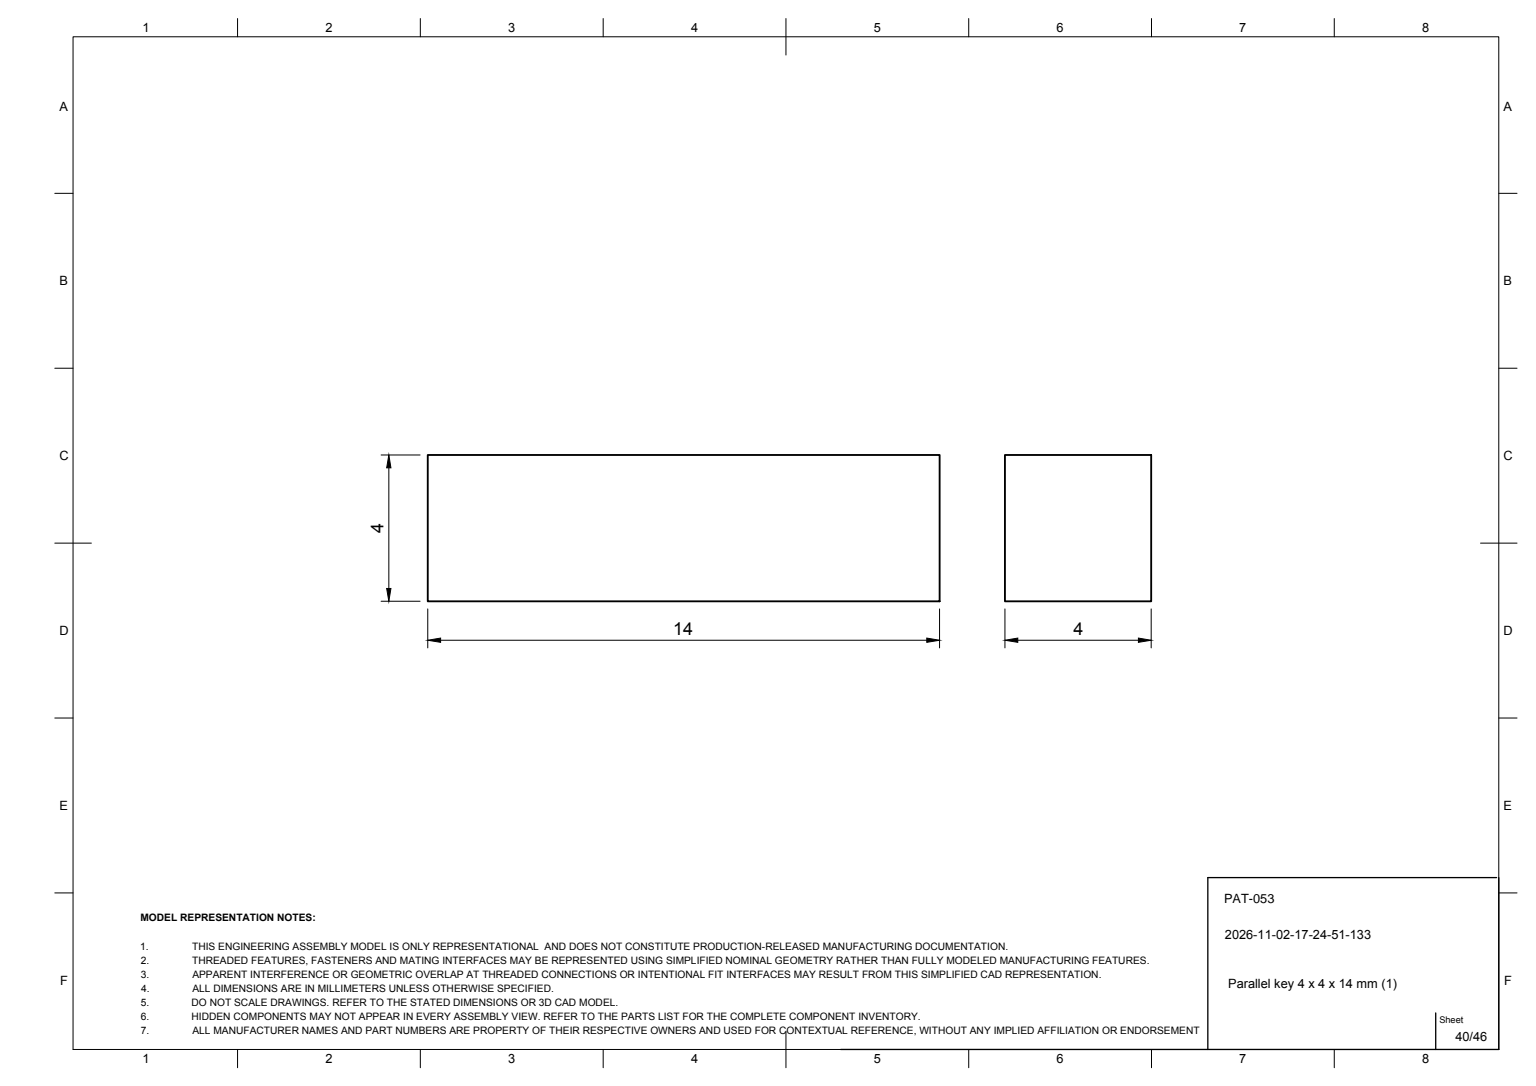
ISO-10303-21;
HEADER;
/* Generated by software containing ST-Developer
 * from STEP Tools, Inc. (www.steptools.com) 
 */

FILE_DESCRIPTION(
/* description */ ('Hand-operated arbor press'),
/* implementation_level */ '2;1');

FILE_NAME(
/* name */ 'Parallel key 4 x 4 x 14 mm (1).step',
/* time_stamp */ '2026-10-28T03:25:25-07:00',
/* author */ (''),
/* organization */ (''),
/* preprocessor_version */ 'ST-DEVELOPER v20.2',
/* originating_system */ 'Autodesk Translation Framework v15.17.0.0',
/* authorisation */ '');

FILE_SCHEMA (('AUTOMOTIVE_DESIGN { 1 0 10303 214 3 1 1 }'));
ENDSEC;

DATA;
#10=MECHANICAL_DESIGN_GEOMETRIC_PRESENTATION_REPRESENTATION('',(#625),#32751);
#534=SHAPE_REPRESENTATION_RELATIONSHIP('SRR','None',#32966,#576);
#576=ADVANCED_BREP_SHAPE_REPRESENTATION('',(#672),#32740);
#625=STYLED_ITEM('',(#33242),#672);
#672=MANIFOLD_SOLID_BREP('Body1',#12524);
#1220=PLANE('',#13866);
#1221=PLANE('',#13867);
#1222=PLANE('',#13868);
#1223=PLANE('',#13869);
#1224=PLANE('',#13870);
#1225=PLANE('',#13871);
#1813=FACE_OUTER_BOUND('',#2643,.T.);
#1814=FACE_OUTER_BOUND('',#2644,.T.);
#1815=FACE_OUTER_BOUND('',#2645,.T.);
#1816=FACE_OUTER_BOUND('',#2646,.T.);
#1817=FACE_OUTER_BOUND('',#2647,.T.);
#1818=FACE_OUTER_BOUND('',#2648,.T.);
#2643=EDGE_LOOP('',(#10860,#10861,#10862,#10863));
#2644=EDGE_LOOP('',(#10864,#10865,#10866,#10867));
#2645=EDGE_LOOP('',(#10868,#10869,#10870,#10871));
#2646=EDGE_LOOP('',(#10872,#10873,#10874,#10875));
#2647=EDGE_LOOP('',(#10876,#10877,#10878,#10879));
#2648=EDGE_LOOP('',(#10880,#10881,#10882,#10883));
#3774=LINE('',#20689,#4945);
#3775=LINE('',#20691,#4946);
#3776=LINE('',#20693,#4947);
#3777=LINE('',#20694,#4948);
#3778=LINE('',#20697,#4949);
#3779=LINE('',#20699,#4950);
#3780=LINE('',#20700,#4951);
#3781=LINE('',#20703,#4952);
#3782=LINE('',#20705,#4953);
#3783=LINE('',#20706,#4954);
#3784=LINE('',#20708,#4955);
#3785=LINE('',#20709,#4956);
#4945=VECTOR('',#16841,1.);
#4946=VECTOR('',#16842,1.);
#4947=VECTOR('',#16843,1.);
#4948=VECTOR('',#16844,1.);
#4949=VECTOR('',#16847,1.);
#4950=VECTOR('',#16848,1.);
#4951=VECTOR('',#16849,1.);
#4952=VECTOR('',#16852,1.);
#4953=VECTOR('',#16853,1.);
#4954=VECTOR('',#16854,1.);
#4955=VECTOR('',#16857,1.);
#4956=VECTOR('',#16858,1.);
#6407=VERTEX_POINT('',#20687);
#6408=VERTEX_POINT('',#20688);
#6409=VERTEX_POINT('',#20690);
#6410=VERTEX_POINT('',#20692);
#6411=VERTEX_POINT('',#20696);
#6412=VERTEX_POINT('',#20698);
#6413=VERTEX_POINT('',#20702);
#6414=VERTEX_POINT('',#20704);
#7933=EDGE_CURVE('',#6407,#6408,#3774,.T.);
#7934=EDGE_CURVE('',#6408,#6409,#3775,.T.);
#7935=EDGE_CURVE('',#6410,#6409,#3776,.T.);
#7936=EDGE_CURVE('',#6407,#6410,#3777,.T.);
#7937=EDGE_CURVE('',#6411,#6407,#3778,.T.);
#7938=EDGE_CURVE('',#6412,#6410,#3779,.T.);
#7939=EDGE_CURVE('',#6411,#6412,#3780,.T.);
#7940=EDGE_CURVE('',#6413,#6411,#3781,.T.);
#7941=EDGE_CURVE('',#6414,#6412,#3782,.T.);
#7942=EDGE_CURVE('',#6413,#6414,#3783,.T.);
#7943=EDGE_CURVE('',#6408,#6413,#3784,.T.);
#7944=EDGE_CURVE('',#6409,#6414,#3785,.T.);
#10860=ORIENTED_EDGE('',*,*,#7933,.T.);
#10861=ORIENTED_EDGE('',*,*,#7934,.T.);
#10862=ORIENTED_EDGE('',*,*,#7935,.F.);
#10863=ORIENTED_EDGE('',*,*,#7936,.F.);
#10864=ORIENTED_EDGE('',*,*,#7937,.T.);
#10865=ORIENTED_EDGE('',*,*,#7936,.T.);
#10866=ORIENTED_EDGE('',*,*,#7938,.F.);
#10867=ORIENTED_EDGE('',*,*,#7939,.F.);
#10868=ORIENTED_EDGE('',*,*,#7940,.T.);
#10869=ORIENTED_EDGE('',*,*,#7939,.T.);
#10870=ORIENTED_EDGE('',*,*,#7941,.F.);
#10871=ORIENTED_EDGE('',*,*,#7942,.F.);
#10872=ORIENTED_EDGE('',*,*,#7943,.T.);
#10873=ORIENTED_EDGE('',*,*,#7942,.T.);
#10874=ORIENTED_EDGE('',*,*,#7944,.F.);
#10875=ORIENTED_EDGE('',*,*,#7934,.F.);
#10876=ORIENTED_EDGE('',*,*,#7944,.T.);
#10877=ORIENTED_EDGE('',*,*,#7941,.T.);
#10878=ORIENTED_EDGE('',*,*,#7938,.T.);
#10879=ORIENTED_EDGE('',*,*,#7935,.T.);
#10880=ORIENTED_EDGE('',*,*,#7943,.F.);
#10881=ORIENTED_EDGE('',*,*,#7933,.F.);
#10882=ORIENTED_EDGE('',*,*,#7937,.F.);
#10883=ORIENTED_EDGE('',*,*,#7940,.F.);
#12322=ADVANCED_FACE('',(#1813),#1220,.T.);
#12323=ADVANCED_FACE('',(#1814),#1221,.T.);
#12324=ADVANCED_FACE('',(#1815),#1222,.T.);
#12325=ADVANCED_FACE('',(#1816),#1223,.T.);
#12326=ADVANCED_FACE('',(#1817),#1224,.T.);
#12327=ADVANCED_FACE('',(#1818),#1225,.F.);
#12524=CLOSED_SHELL('',(#12322,#12323,#12324,#12325,#12326,#12327));
#13865=AXIS2_PLACEMENT_3D('',#20685,#16837,#16838);
#13866=AXIS2_PLACEMENT_3D('',#20686,#16839,#16840);
#13867=AXIS2_PLACEMENT_3D('',#20695,#16845,#16846);
#13868=AXIS2_PLACEMENT_3D('',#20701,#16850,#16851);
#13869=AXIS2_PLACEMENT_3D('',#20707,#16855,#16856);
#13870=AXIS2_PLACEMENT_3D('',#20710,#16859,#16860);
#13871=AXIS2_PLACEMENT_3D('',#20711,#16861,#16862);
#16837=DIRECTION('axis',(0.,0.,1.));
#16838=DIRECTION('refdir',(1.,0.,0.));
#16839=DIRECTION('center_axis',(0.,1.,0.));
#16840=DIRECTION('ref_axis',(-1.,0.,0.));
#16841=DIRECTION('',(-1.,0.,0.));
#16842=DIRECTION('',(0.,0.,1.));
#16843=DIRECTION('',(-1.,0.,0.));
#16844=DIRECTION('',(0.,0.,1.));
#16845=DIRECTION('center_axis',(1.,0.,0.));
#16846=DIRECTION('ref_axis',(0.,1.,0.));
#16847=DIRECTION('',(0.,1.,0.));
#16848=DIRECTION('',(0.,1.,0.));
#16849=DIRECTION('',(0.,0.,1.));
#16850=DIRECTION('center_axis',(0.,-1.,0.));
#16851=DIRECTION('ref_axis',(1.,0.,0.));
#16852=DIRECTION('',(1.,0.,0.));
#16853=DIRECTION('',(1.,0.,0.));
#16854=DIRECTION('',(0.,0.,1.));
#16855=DIRECTION('center_axis',(-1.,0.,0.));
#16856=DIRECTION('ref_axis',(0.,-1.,0.));
#16857=DIRECTION('',(0.,-1.,0.));
#16858=DIRECTION('',(0.,-1.,0.));
#16859=DIRECTION('center_axis',(0.,0.,1.));
#16860=DIRECTION('ref_axis',(1.,0.,0.));
#16861=DIRECTION('center_axis',(0.,0.,1.));
#16862=DIRECTION('ref_axis',(1.,0.,0.));
#20685=CARTESIAN_POINT('',(0.,0.,0.));
#20686=CARTESIAN_POINT('Origin',(-2.5,6.9,19.8));
#20687=CARTESIAN_POINT('',(-2.5,6.9,19.8));
#20688=CARTESIAN_POINT('',(-2.9,6.9,19.8));
#20689=CARTESIAN_POINT('',(-2.5,6.9,19.8));
#20690=CARTESIAN_POINT('',(-2.9,6.9,20.2));
#20691=CARTESIAN_POINT('',(-2.9,6.9,19.8));
#20692=CARTESIAN_POINT('',(-2.5,6.9,20.2));
#20693=CARTESIAN_POINT('',(-2.5,6.9,20.2));
#20694=CARTESIAN_POINT('',(-2.5,6.9,19.8));
#20695=CARTESIAN_POINT('Origin',(-2.5,5.5,19.8));
#20696=CARTESIAN_POINT('',(-2.5,5.5,19.8));
#20697=CARTESIAN_POINT('',(-2.5,5.5,19.8));
#20698=CARTESIAN_POINT('',(-2.5,5.5,20.2));
#20699=CARTESIAN_POINT('',(-2.5,5.5,20.2));
#20700=CARTESIAN_POINT('',(-2.5,5.5,19.8));
#20701=CARTESIAN_POINT('Origin',(-2.9,5.5,19.8));
#20702=CARTESIAN_POINT('',(-2.9,5.5,19.8));
#20703=CARTESIAN_POINT('',(-2.9,5.5,19.8));
#20704=CARTESIAN_POINT('',(-2.9,5.5,20.2));
#20705=CARTESIAN_POINT('',(-2.9,5.5,20.2));
#20706=CARTESIAN_POINT('',(-2.9,5.5,19.8));
#20707=CARTESIAN_POINT('Origin',(-2.9,6.9,19.8));
#20708=CARTESIAN_POINT('',(-2.9,6.9,19.8));
#20709=CARTESIAN_POINT('',(-2.9,6.9,20.2));
#20710=CARTESIAN_POINT('Origin',(-2.7,6.2,20.2));
#20711=CARTESIAN_POINT('Origin',(-2.7,6.2,19.8));
#32691=UNCERTAINTY_MEASURE_WITH_UNIT(LENGTH_MEASURE(0.001),#32752,
'DISTANCE_ACCURACY_VALUE',
'Maximum model space distance between geometric entities at asserted c
onnectivities');
#32702=UNCERTAINTY_MEASURE_WITH_UNIT(LENGTH_MEASURE(0.001),#32752,
'DISTANCE_ACCURACY_VALUE',
'Maximum model space distance between geometric entities at asserted c
onnectivities');
#32740=(
GEOMETRIC_REPRESENTATION_CONTEXT(3)
GLOBAL_UNCERTAINTY_ASSIGNED_CONTEXT((#32691))
GLOBAL_UNIT_ASSIGNED_CONTEXT((#32752,#32754,#32755))
REPRESENTATION_CONTEXT('','3D')
);
#32751=(
GEOMETRIC_REPRESENTATION_CONTEXT(3)
GLOBAL_UNCERTAINTY_ASSIGNED_CONTEXT((#32702))
GLOBAL_UNIT_ASSIGNED_CONTEXT((#32752,#32754,#32755))
REPRESENTATION_CONTEXT('','3D')
);
#32752=(
LENGTH_UNIT()
NAMED_UNIT(*)
SI_UNIT(.CENTI.,.METRE.)
);
#32754=(
NAMED_UNIT(*)
PLANE_ANGLE_UNIT()
SI_UNIT($,.RADIAN.)
);
#32755=(
NAMED_UNIT(*)
SI_UNIT($,.STERADIAN.)
SOLID_ANGLE_UNIT()
);
#32793=SHAPE_DEFINITION_REPRESENTATION(#32850,#32966);
#32850=PRODUCT_DEFINITION_SHAPE('',$,#33015);
#32966=SHAPE_REPRESENTATION('',(#13865),#32740);
#32977=PRODUCT_DEFINITION_CONTEXT('part definition',#33123,'design');
#33015=PRODUCT_DEFINITION('Parallel key 4 x 4 x 14 mm (1)',
'Parallel key 4 x 4 x 14 mm (1)',#33063,#32977);
#33063=PRODUCT_DEFINITION_FORMATION('',$,#33162);
#33123=APPLICATION_CONTEXT(
'Core Data for Automotive Mechanical Design Process');
#33124=PRODUCT_CONTEXT('part definition',#33123,'mechanical');
#33162=PRODUCT('Parallel key 4 x 4 x 14 mm (1)',
'Parallel key 4 x 4 x 14 mm (1)','Parallel key 4 x 4 x 14 mm (1)',(#33124));
#33236=COLOUR_RGB('Grey',0.48,0.52,0.57);
#33237=FILL_AREA_STYLE_COLOUR('',#33236);
#33238=FILL_AREA_STYLE('',(#33237));
#33239=SURFACE_STYLE_FILL_AREA(#33238);
#33240=SURFACE_SIDE_STYLE('',(#33239));
#33241=SURFACE_STYLE_USAGE(.BOTH.,#33240);
#33242=PRESENTATION_STYLE_ASSIGNMENT((#33241));
ENDSEC;
END-ISO-10303-21;
